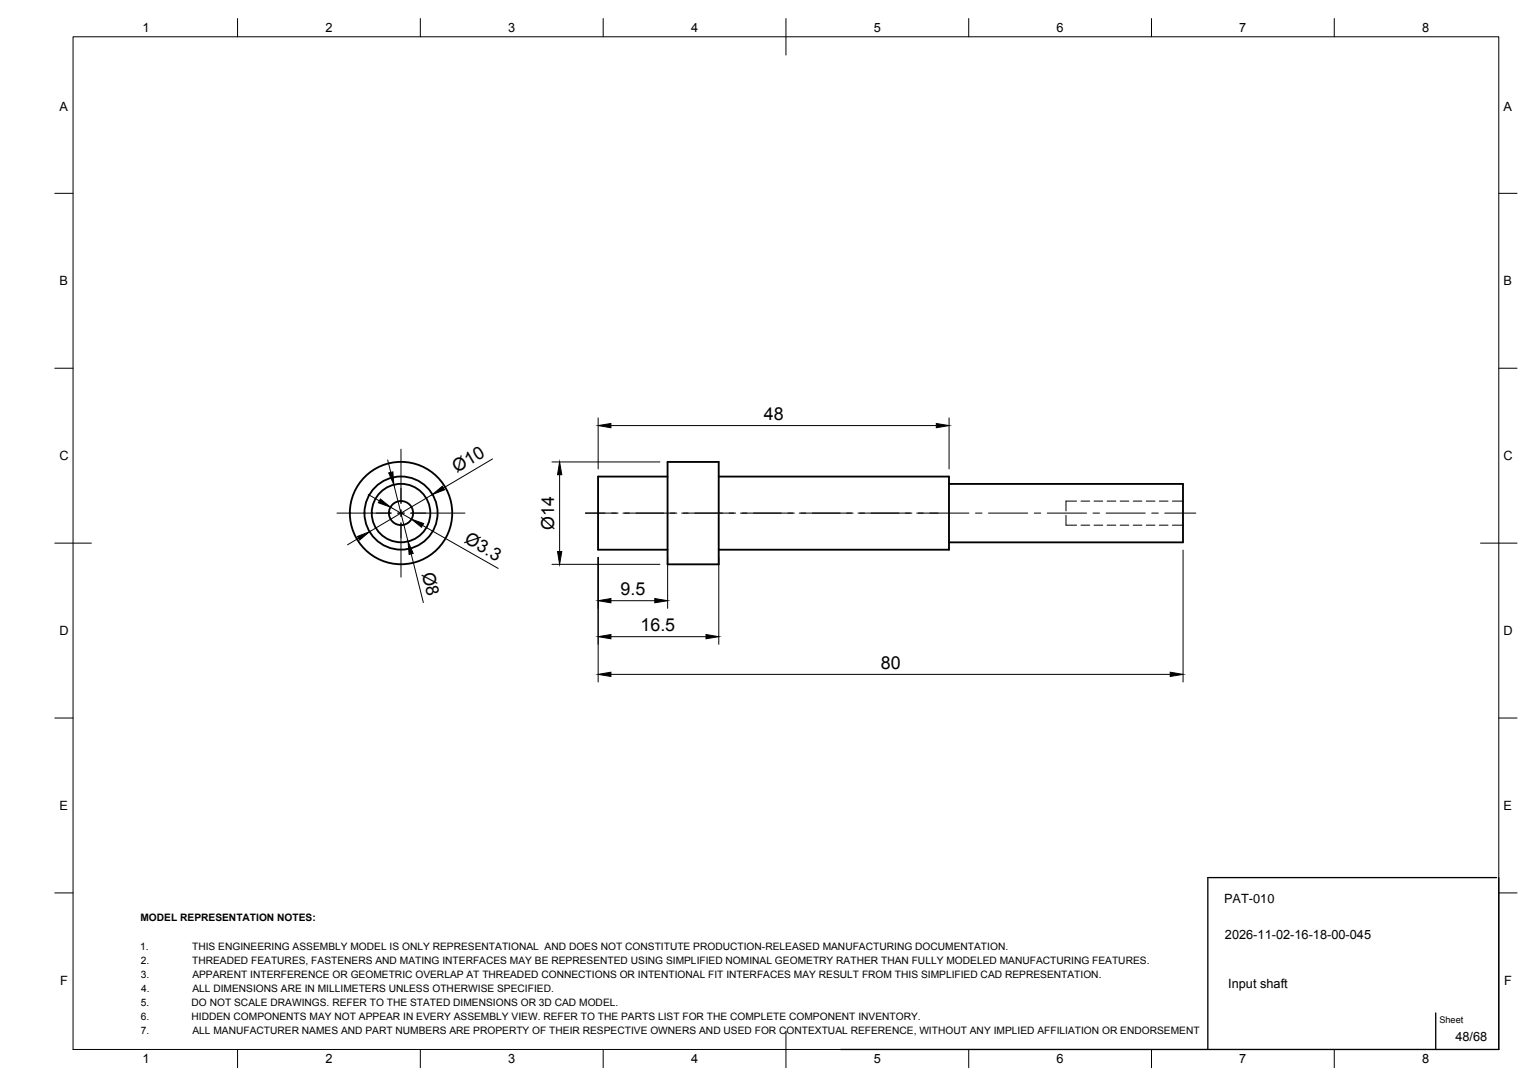
ISO-10303-21;
HEADER;
/* Generated by software containing ST-Developer
 * from STEP Tools, Inc. (www.steptools.com) 
 */

FILE_DESCRIPTION(
/* description */ ('Belt conveyor head drive unit'),
/* implementation_level */ '2;1');

FILE_NAME(
/* name */ 'Input shaft.step',
/* time_stamp */ '2026-10-28T03:26:19-07:00',
/* author */ (''),
/* organization */ (''),
/* preprocessor_version */ 'ST-DEVELOPER v20.2',
/* originating_system */ 'Autodesk Translation Framework v15.17.0.0',
/* authorisation */ '');

FILE_SCHEMA (('AUTOMOTIVE_DESIGN { 1 0 10303 214 3 1 1 }'));
ENDSEC;

DATA;
#10=MECHANICAL_DESIGN_GEOMETRIC_PRESENTATION_REPRESENTATION('',(#907),#27069);
#753=SHAPE_REPRESENTATION_RELATIONSHIP('SRR','None',#27401,#822);
#822=ADVANCED_BREP_SHAPE_REPRESENTATION('',(#988),#27043);
#907=STYLED_ITEM('',(#27797),#988);
#988=MANIFOLD_SOLID_BREP('Body1',#13776);
#1205=FACE_BOUND('',#3143,.T.);
#1206=FACE_BOUND('',#3145,.T.);
#1207=FACE_BOUND('',#3150,.T.);
#1208=FACE_BOUND('',#3154,.T.);
#1541=PLANE('',#15641);
#1542=PLANE('',#15642);
#1543=PLANE('',#15645);
#1544=PLANE('',#15654);
#1545=PLANE('',#15657);
#1546=PLANE('',#15658);
#2147=FACE_OUTER_BOUND('',#3140,.T.);
#2148=FACE_OUTER_BOUND('',#3141,.T.);
#2149=FACE_OUTER_BOUND('',#3142,.T.);
#2150=FACE_OUTER_BOUND('',#3144,.T.);
#2151=FACE_OUTER_BOUND('',#3146,.T.);
#2152=FACE_OUTER_BOUND('',#3147,.T.);
#2153=FACE_OUTER_BOUND('',#3148,.T.);
#2154=FACE_OUTER_BOUND('',#3149,.T.);
#2155=FACE_OUTER_BOUND('',#3151,.T.);
#2156=FACE_OUTER_BOUND('',#3152,.T.);
#2157=FACE_OUTER_BOUND('',#3153,.T.);
#3140=EDGE_LOOP('',(#11160,#11161,#11162,#11163));
#3141=EDGE_LOOP('',(#11164));
#3142=EDGE_LOOP('',(#11165));
#3143=EDGE_LOOP('',(#11166));
#3144=EDGE_LOOP('',(#11167));
#3145=EDGE_LOOP('',(#11168));
#3146=EDGE_LOOP('',(#11169,#11170,#11171,#11172));
#3147=EDGE_LOOP('',(#11173,#11174,#11175,#11176));
#3148=EDGE_LOOP('',(#11177,#11178,#11179,#11180));
#3149=EDGE_LOOP('',(#11181));
#3150=EDGE_LOOP('',(#11182));
#3151=EDGE_LOOP('',(#11183,#11184,#11185,#11186));
#3152=EDGE_LOOP('',(#11187));
#3153=EDGE_LOOP('',(#11188));
#3154=EDGE_LOOP('',(#11189));
#4044=LINE('',#24446,#4836);
#4045=LINE('',#24460,#4837);
#4046=LINE('',#24463,#4838);
#4047=LINE('',#24469,#4839);
#4048=LINE('',#24475,#4840);
#4836=VECTOR('',#19136,0.165);
#4837=VECTOR('',#19155,0.7);
#4838=VECTOR('',#19158,0.5);
#4839=VECTOR('',#19165,0.4);
#4840=VECTOR('',#19174,0.5);
#5581=CIRCLE('',#15639,0.165);
#5582=CIRCLE('',#15640,0.165);
#5583=CIRCLE('',#15643,0.7);
#5584=CIRCLE('',#15644,0.5);
#5585=CIRCLE('',#15646,0.7);
#5586=CIRCLE('',#15647,0.5);
#5587=CIRCLE('',#15650,0.5);
#5588=CIRCLE('',#15652,0.4);
#5589=CIRCLE('',#15653,0.4);
#5590=CIRCLE('',#15656,0.5);
#6707=VERTEX_POINT('',#24443);
#6708=VERTEX_POINT('',#24445);
#6709=VERTEX_POINT('',#24450);
#6710=VERTEX_POINT('',#24452);
#6711=VERTEX_POINT('',#24455);
#6712=VERTEX_POINT('',#24457);
#6713=VERTEX_POINT('',#24462);
#6714=VERTEX_POINT('',#24466);
#6715=VERTEX_POINT('',#24468);
#6716=VERTEX_POINT('',#24473);
#8272=EDGE_CURVE('',#6707,#6707,#5581,.T.);
#8273=EDGE_CURVE('',#6707,#6708,#4044,.T.);
#8274=EDGE_CURVE('',#6708,#6708,#5582,.T.);
#8275=EDGE_CURVE('',#6709,#6709,#5583,.T.);
#8276=EDGE_CURVE('',#6710,#6710,#5584,.T.);
#8277=EDGE_CURVE('',#6711,#6711,#5585,.T.);
#8278=EDGE_CURVE('',#6712,#6712,#5586,.T.);
#8279=EDGE_CURVE('',#6709,#6711,#4045,.T.);
#8280=EDGE_CURVE('',#6712,#6713,#4046,.T.);
#8281=EDGE_CURVE('',#6713,#6713,#5587,.T.);
#8282=EDGE_CURVE('',#6714,#6714,#5588,.T.);
#8283=EDGE_CURVE('',#6714,#6715,#4047,.T.);
#8284=EDGE_CURVE('',#6715,#6715,#5589,.T.);
#8285=EDGE_CURVE('',#6716,#6716,#5590,.T.);
#8286=EDGE_CURVE('',#6716,#6710,#4048,.T.);
#11160=ORIENTED_EDGE('',*,*,#8272,.F.);
#11161=ORIENTED_EDGE('',*,*,#8273,.T.);
#11162=ORIENTED_EDGE('',*,*,#8274,.T.);
#11163=ORIENTED_EDGE('',*,*,#8273,.F.);
#11164=ORIENTED_EDGE('',*,*,#8274,.F.);
#11165=ORIENTED_EDGE('',*,*,#8275,.T.);
#11166=ORIENTED_EDGE('',*,*,#8276,.F.);
#11167=ORIENTED_EDGE('',*,*,#8277,.F.);
#11168=ORIENTED_EDGE('',*,*,#8278,.F.);
#11169=ORIENTED_EDGE('',*,*,#8275,.F.);
#11170=ORIENTED_EDGE('',*,*,#8279,.T.);
#11171=ORIENTED_EDGE('',*,*,#8277,.T.);
#11172=ORIENTED_EDGE('',*,*,#8279,.F.);
#11173=ORIENTED_EDGE('',*,*,#8278,.T.);
#11174=ORIENTED_EDGE('',*,*,#8280,.T.);
#11175=ORIENTED_EDGE('',*,*,#8281,.T.);
#11176=ORIENTED_EDGE('',*,*,#8280,.F.);
#11177=ORIENTED_EDGE('',*,*,#8282,.F.);
#11178=ORIENTED_EDGE('',*,*,#8283,.T.);
#11179=ORIENTED_EDGE('',*,*,#8284,.T.);
#11180=ORIENTED_EDGE('',*,*,#8283,.F.);
#11181=ORIENTED_EDGE('',*,*,#8284,.F.);
#11182=ORIENTED_EDGE('',*,*,#8272,.T.);
#11183=ORIENTED_EDGE('',*,*,#8285,.F.);
#11184=ORIENTED_EDGE('',*,*,#8286,.T.);
#11185=ORIENTED_EDGE('',*,*,#8276,.T.);
#11186=ORIENTED_EDGE('',*,*,#8286,.F.);
#11187=ORIENTED_EDGE('',*,*,#8285,.T.);
#11188=ORIENTED_EDGE('',*,*,#8281,.F.);
#11189=ORIENTED_EDGE('',*,*,#8282,.T.);
#12724=CYLINDRICAL_SURFACE('',#15638,0.165);
#12725=CYLINDRICAL_SURFACE('',#15648,0.7);
#12726=CYLINDRICAL_SURFACE('',#15649,0.5);
#12727=CYLINDRICAL_SURFACE('',#15651,0.4);
#12728=CYLINDRICAL_SURFACE('',#15655,0.5);
#13426=ADVANCED_FACE('',(#2147),#12724,.F.);
#13427=ADVANCED_FACE('',(#2148),#1541,.F.);
#13428=ADVANCED_FACE('',(#2149,#1205),#1542,.T.);
#13429=ADVANCED_FACE('',(#2150,#1206),#1543,.F.);
#13430=ADVANCED_FACE('',(#2151),#12725,.T.);
#13431=ADVANCED_FACE('',(#2152),#12726,.T.);
#13432=ADVANCED_FACE('',(#2153),#12727,.T.);
#13433=ADVANCED_FACE('',(#2154,#1207),#1544,.F.);
#13434=ADVANCED_FACE('',(#2155),#12728,.T.);
#13435=ADVANCED_FACE('',(#2156),#1545,.T.);
#13436=ADVANCED_FACE('',(#2157,#1208),#1546,.F.);
#13776=CLOSED_SHELL('',(#13426,#13427,#13428,#13429,#13430,#13431,#13432,
#13433,#13434,#13435,#13436));
#15637=AXIS2_PLACEMENT_3D('',#24441,#19130,#19131);
#15638=AXIS2_PLACEMENT_3D('',#24442,#19132,#19133);
#15639=AXIS2_PLACEMENT_3D('',#24444,#19134,#19135);
#15640=AXIS2_PLACEMENT_3D('',#24447,#19137,#19138);
#15641=AXIS2_PLACEMENT_3D('',#24448,#19139,#19140);
#15642=AXIS2_PLACEMENT_3D('',#24449,#19141,#19142);
#15643=AXIS2_PLACEMENT_3D('',#24451,#19143,#19144);
#15644=AXIS2_PLACEMENT_3D('',#24453,#19145,#19146);
#15645=AXIS2_PLACEMENT_3D('',#24454,#19147,#19148);
#15646=AXIS2_PLACEMENT_3D('',#24456,#19149,#19150);
#15647=AXIS2_PLACEMENT_3D('',#24458,#19151,#19152);
#15648=AXIS2_PLACEMENT_3D('',#24459,#19153,#19154);
#15649=AXIS2_PLACEMENT_3D('',#24461,#19156,#19157);
#15650=AXIS2_PLACEMENT_3D('',#24464,#19159,#19160);
#15651=AXIS2_PLACEMENT_3D('',#24465,#19161,#19162);
#15652=AXIS2_PLACEMENT_3D('',#24467,#19163,#19164);
#15653=AXIS2_PLACEMENT_3D('',#24470,#19166,#19167);
#15654=AXIS2_PLACEMENT_3D('',#24471,#19168,#19169);
#15655=AXIS2_PLACEMENT_3D('',#24472,#19170,#19171);
#15656=AXIS2_PLACEMENT_3D('',#24474,#19172,#19173);
#15657=AXIS2_PLACEMENT_3D('',#24476,#19175,#19176);
#15658=AXIS2_PLACEMENT_3D('',#24477,#19177,#19178);
#19130=DIRECTION('axis',(0.,0.,1.));
#19131=DIRECTION('refdir',(1.,0.,0.));
#19132=DIRECTION('center_axis',(0.,1.,0.));
#19133=DIRECTION('ref_axis',(1.,0.,0.));
#19134=DIRECTION('center_axis',(0.,1.,0.));
#19135=DIRECTION('ref_axis',(1.,0.,0.));
#19136=DIRECTION('',(0.,1.,0.));
#19137=DIRECTION('center_axis',(0.,1.,0.));
#19138=DIRECTION('ref_axis',(1.,0.,0.));
#19139=DIRECTION('center_axis',(0.,1.,0.));
#19140=DIRECTION('ref_axis',(1.,0.,0.));
#19141=DIRECTION('center_axis',(0.,1.,0.));
#19142=DIRECTION('ref_axis',(1.,0.,0.));
#19143=DIRECTION('center_axis',(0.,1.,0.));
#19144=DIRECTION('ref_axis',(1.,0.,0.));
#19145=DIRECTION('center_axis',(0.,1.,0.));
#19146=DIRECTION('ref_axis',(1.,0.,0.));
#19147=DIRECTION('center_axis',(0.,1.,0.));
#19148=DIRECTION('ref_axis',(1.,0.,0.));
#19149=DIRECTION('center_axis',(0.,1.,0.));
#19150=DIRECTION('ref_axis',(1.,0.,0.));
#19151=DIRECTION('center_axis',(0.,-1.,0.));
#19152=DIRECTION('ref_axis',(1.,0.,0.));
#19153=DIRECTION('center_axis',(0.,1.,0.));
#19154=DIRECTION('ref_axis',(1.,0.,0.));
#19155=DIRECTION('',(0.,-1.,0.));
#19156=DIRECTION('center_axis',(0.,1.,0.));
#19157=DIRECTION('ref_axis',(1.,0.,0.));
#19158=DIRECTION('',(0.,-1.,0.));
#19159=DIRECTION('center_axis',(0.,1.,0.));
#19160=DIRECTION('ref_axis',(1.,0.,0.));
#19161=DIRECTION('center_axis',(0.,1.,0.));
#19162=DIRECTION('ref_axis',(1.,0.,0.));
#19163=DIRECTION('center_axis',(0.,1.,0.));
#19164=DIRECTION('ref_axis',(1.,0.,0.));
#19165=DIRECTION('',(0.,-1.,0.));
#19166=DIRECTION('center_axis',(0.,1.,0.));
#19167=DIRECTION('ref_axis',(1.,0.,0.));
#19168=DIRECTION('center_axis',(0.,1.,0.));
#19169=DIRECTION('ref_axis',(1.,0.,0.));
#19170=DIRECTION('center_axis',(0.,1.,0.));
#19171=DIRECTION('ref_axis',(1.,0.,0.));
#19172=DIRECTION('center_axis',(0.,1.,0.));
#19173=DIRECTION('ref_axis',(1.,0.,0.));
#19174=DIRECTION('',(0.,-1.,0.));
#19175=DIRECTION('center_axis',(0.,1.,0.));
#19176=DIRECTION('ref_axis',(1.,0.,0.));
#19177=DIRECTION('center_axis',(0.,1.,0.));
#19178=DIRECTION('ref_axis',(1.,0.,0.));
#24441=CARTESIAN_POINT('',(0.,0.,0.));
#24442=CARTESIAN_POINT('Origin',(0.,-5.1,7.));
#24443=CARTESIAN_POINT('',(-0.165,-5.,7.));
#24444=CARTESIAN_POINT('Origin',(0.,-5.,7.));
#24445=CARTESIAN_POINT('',(-0.165,-3.4,7.));
#24446=CARTESIAN_POINT('',(-0.165,-5.1,7.));
#24447=CARTESIAN_POINT('Origin',(0.,-3.4,7.));
#24448=CARTESIAN_POINT('Origin',(0.,-3.4,7.));
#24449=CARTESIAN_POINT('Origin',(0.,2.05,7.));
#24450=CARTESIAN_POINT('',(-0.7,2.05,7.));
#24451=CARTESIAN_POINT('Origin',(0.,2.05,7.));
#24452=CARTESIAN_POINT('',(-0.5,2.05,7.));
#24453=CARTESIAN_POINT('Origin',(0.,2.05,7.));
#24454=CARTESIAN_POINT('Origin',(0.,1.35,7.));
#24455=CARTESIAN_POINT('',(-0.7,1.35,7.));
#24456=CARTESIAN_POINT('Origin',(0.,1.35,7.));
#24457=CARTESIAN_POINT('',(-0.5,1.35,7.));
#24458=CARTESIAN_POINT('Origin',(0.,1.35,7.));
#24459=CARTESIAN_POINT('Origin',(0.,1.35,7.));
#24460=CARTESIAN_POINT('',(-0.7,1.35,7.));
#24461=CARTESIAN_POINT('Origin',(0.,-1.8,7.));
#24462=CARTESIAN_POINT('',(-0.5,-1.8,7.));
#24463=CARTESIAN_POINT('',(-0.5,-1.8,7.));
#24464=CARTESIAN_POINT('Origin',(0.,-1.8,7.));
#24465=CARTESIAN_POINT('Origin',(0.,-5.,7.));
#24466=CARTESIAN_POINT('',(-0.4,-1.8,7.));
#24467=CARTESIAN_POINT('Origin',(0.,-1.8,7.));
#24468=CARTESIAN_POINT('',(-0.4,-5.,7.));
#24469=CARTESIAN_POINT('',(-0.4,-5.,7.));
#24470=CARTESIAN_POINT('Origin',(0.,-5.,7.));
#24471=CARTESIAN_POINT('Origin',(0.,-5.,7.));
#24472=CARTESIAN_POINT('Origin',(0.,-1.8,7.));
#24473=CARTESIAN_POINT('',(-0.5,3.,7.));
#24474=CARTESIAN_POINT('Origin',(0.,3.,7.));
#24475=CARTESIAN_POINT('',(-0.5,-1.8,7.));
#24476=CARTESIAN_POINT('Origin',(0.,3.,7.));
#24477=CARTESIAN_POINT('Origin',(0.,-1.8,7.));
#26966=UNCERTAINTY_MEASURE_WITH_UNIT(LENGTH_MEASURE(0.001),#27070,
'DISTANCE_ACCURACY_VALUE',
'Maximum model space distance between geometric entities at asserted c
onnectivities');
#26992=UNCERTAINTY_MEASURE_WITH_UNIT(LENGTH_MEASURE(0.001),#27070,
'DISTANCE_ACCURACY_VALUE',
'Maximum model space distance between geometric entities at asserted c
onnectivities');
#27043=(
GEOMETRIC_REPRESENTATION_CONTEXT(3)
GLOBAL_UNCERTAINTY_ASSIGNED_CONTEXT((#26966))
GLOBAL_UNIT_ASSIGNED_CONTEXT((#27070,#27072,#27073))
REPRESENTATION_CONTEXT('','3D')
);
#27069=(
GEOMETRIC_REPRESENTATION_CONTEXT(3)
GLOBAL_UNCERTAINTY_ASSIGNED_CONTEXT((#26992))
GLOBAL_UNIT_ASSIGNED_CONTEXT((#27070,#27072,#27073))
REPRESENTATION_CONTEXT('','3D')
);
#27070=(
LENGTH_UNIT()
NAMED_UNIT(*)
SI_UNIT(.CENTI.,.METRE.)
);
#27072=(
NAMED_UNIT(*)
PLANE_ANGLE_UNIT()
SI_UNIT($,.RADIAN.)
);
#27073=(
NAMED_UNIT(*)
SI_UNIT($,.STERADIAN.)
SOLID_ANGLE_UNIT()
);
#27124=SHAPE_DEFINITION_REPRESENTATION(#27212,#27401);
#27212=PRODUCT_DEFINITION_SHAPE('',$,#27478);
#27401=SHAPE_REPRESENTATION('',(#15637),#27043);
#27427=PRODUCT_DEFINITION_CONTEXT('part definition',#27657,'design');
#27478=PRODUCT_DEFINITION('Input shaft','Input shaft',#27554,#27427);
#27554=PRODUCT_DEFINITION_FORMATION('',$,#27709);
#27657=APPLICATION_CONTEXT(
'Core Data for Automotive Mechanical Design Process');
#27658=PRODUCT_CONTEXT('part definition',#27657,'mechanical');
#27709=PRODUCT('Input shaft','Input shaft','Input shaft',(#27658));
#27791=COLOUR_RGB('Grey',0.48,0.52,0.57);
#27792=FILL_AREA_STYLE_COLOUR('',#27791);
#27793=FILL_AREA_STYLE('',(#27792));
#27794=SURFACE_STYLE_FILL_AREA(#27793);
#27795=SURFACE_SIDE_STYLE('',(#27794));
#27796=SURFACE_STYLE_USAGE(.BOTH.,#27795);
#27797=PRESENTATION_STYLE_ASSIGNMENT((#27796));
ENDSEC;
END-ISO-10303-21;
